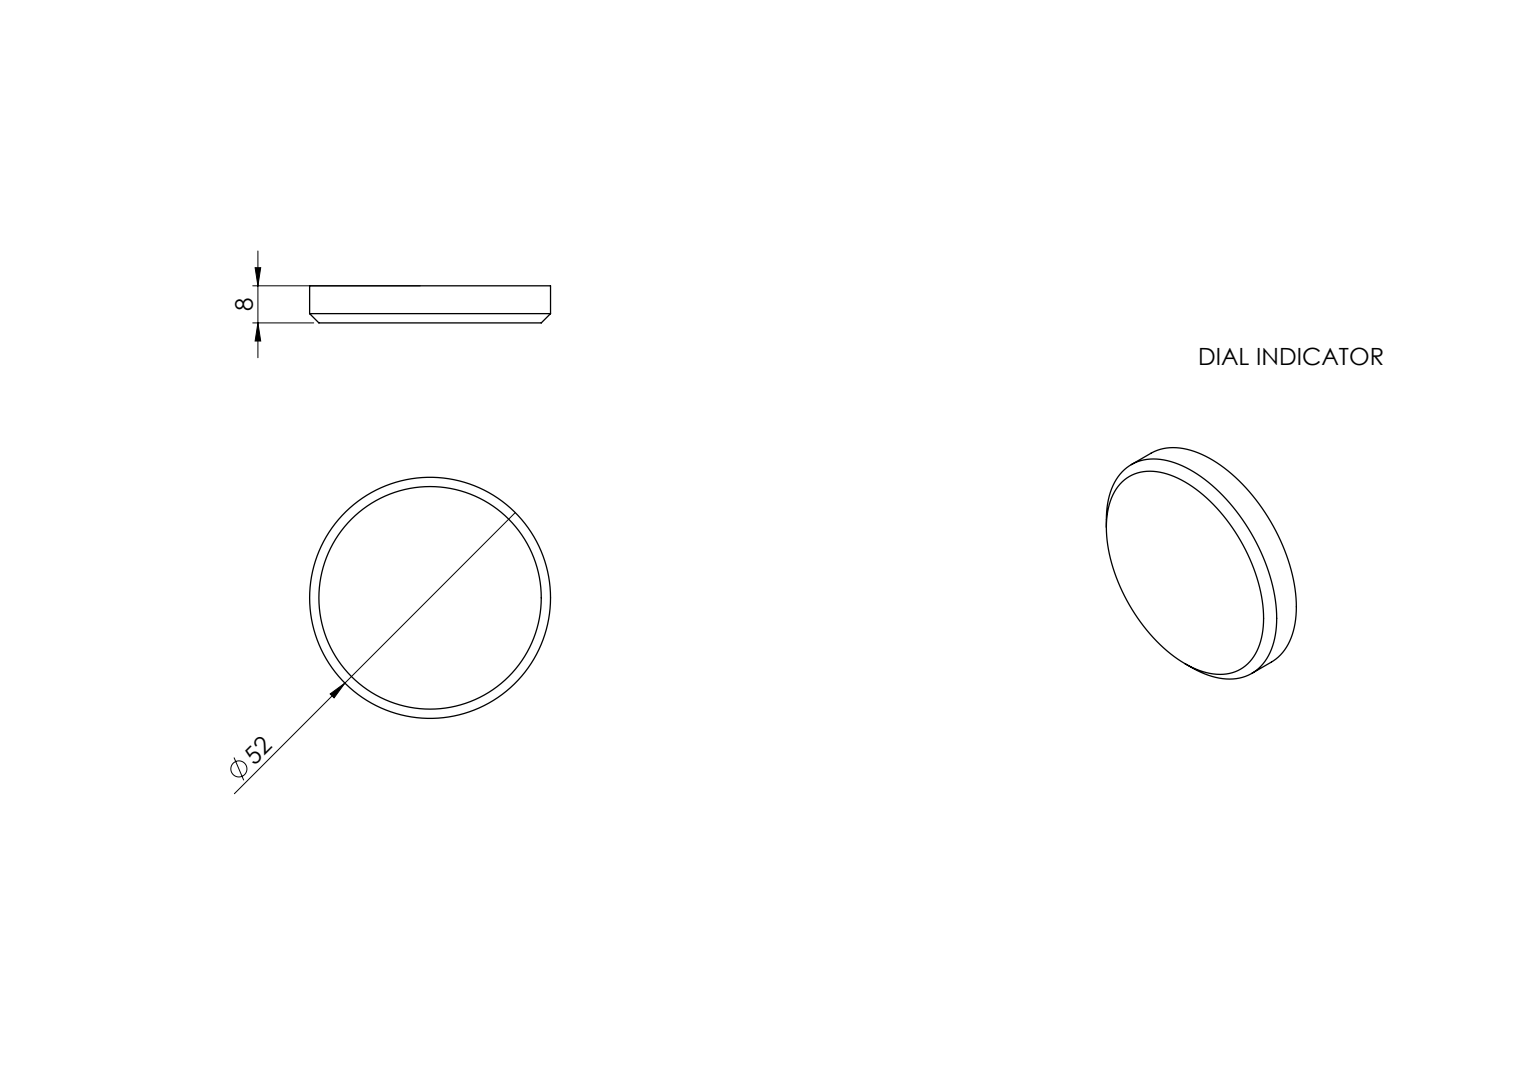
ISO-10303-21;
HEADER;
FILE_DESCRIPTION (('STEP AP214'),
    '1' );
FILE_NAME ('dial indicator.step',
    '2026-10-27T04:40:18',
    ( '' ),
    ( '' ),
    'SwSTEP 2.0',
    'SolidWorks 2026',
    '' );
FILE_SCHEMA (( 'AUTOMOTIVE_DESIGN' ));
ENDSEC;

DATA;
#6=ADVANCED_FACE ( 'NONE', ( #7611 ), #3122, .F. ) ;
#12=DIRECTION ( 'NONE',  ( -1.000000000000000000, 0.000000000000000000, 0.000000000000000000 ) ) ;
#28=DIRECTION ( 'NONE',  ( -1.000000000000000000, 0.000000000000000000, 0.000000000000000000 ) ) ;
#30=LINE ( 'NONE', #3412, #7519 ) ;
#144=CIRCLE ( 'NONE', #2107, 1.000000000000000888 ) ;
#231=DIRECTION ( 'NONE',  ( -1.000000000000000000, 0.000000000000000000, 0.000000000000000000 ) ) ;
#250=DIRECTION ( 'NONE',  ( 1.000000000000000000, 0.000000000000000000, 0.000000000000000000 ) ) ;
#266=DIRECTION ( 'NONE',  ( -0.000000000000000000, -0.000000000000000000, -1.000000000000000000 ) ) ;
#268=DIRECTION ( 'NONE',  ( -1.000000000000000000, 0.000000000000000000, 0.000000000000000000 ) ) ;
#325=EDGE_LOOP ( 'NONE', ( #10518, #10319, #10166, #3050 ) ) ;
#332=LINE ( 'NONE', #9669, #6281 ) ;
#361=ORIENTED_EDGE ( 'NONE', *, *, #10949, .T. ) ;
#401=DIRECTION ( 'NONE',  ( -1.000000000000000000, 0.000000000000000000, 0.000000000000000000 ) ) ;
#435=SURFACE_STYLE_USAGE ( .BOTH. , #2987 ) ;
#461=EDGE_LOOP ( 'NONE', ( #7760, #1425, #10364, #3402 ) ) ;
#484=VERTEX_POINT ( 'NONE', #2961 ) ;
#495=ORIENTED_EDGE ( 'NONE', *, *, #4274, .T. ) ;
#501=CARTESIAN_POINT ( 'NONE',  ( -78.99999999999998579, 11.49999999999999645, 8.000000000000000000 ) ) ;
#506=VERTEX_POINT ( 'NONE', #4670 ) ;
#524=CIRCLE ( 'NONE', #4765, 25.99999999999999645 ) ;
#539=( GEOMETRIC_REPRESENTATION_CONTEXT ( 3 ) GLOBAL_UNCERTAINTY_ASSIGNED_CONTEXT ( ( #6697 ) ) GLOBAL_UNIT_ASSIGNED_CONTEXT ( ( #8208, #6320, #9818 ) ) REPRESENTATION_CONTEXT ( 'NONE', 'WORKASPACE' ) );
#650=( NAMED_UNIT ( * ) PLANE_ANGLE_UNIT ( ) SI_UNIT ( $, .RADIAN. ) );
#658=EDGE_CURVE ( 'NONE', #5256, #1211, #1641, .T. ) ;
#715=ORIENTED_EDGE ( 'NONE', *, *, #4832, .T. ) ;
#780=DIRECTION ( 'NONE',  ( -1.000000000000000000, 0.000000000000000000, 0.000000000000000000 ) ) ;
#782=DIRECTION ( 'NONE',  ( 1.000000000000000000, 0.000000000000000000, 0.000000000000000000 ) ) ;
#839=EDGE_LOOP ( 'NONE', ( #2453, #10131 ) ) ;
#846=DIRECTION ( 'NONE',  ( -0.000000000000000000, -0.000000000000000000, -1.000000000000000000 ) ) ;
#905=AXIS2_PLACEMENT_3D ( 'NONE', #10068, #7575, #3243 ) ;
#911=ADVANCED_FACE ( 'NONE', ( #5426 ), #6787, .F. ) ;
#932=PRODUCT_DEFINITION ( 'UNKNOWN', '', #1061, #2065 ) ;
#973=EDGE_LOOP ( 'NONE', ( #9490, #7582 ) ) ;
#984=LINE ( 'NONE', #3485, #6922 ) ;
#1013=ORIENTED_EDGE ( 'NONE', *, *, #2371, .T. ) ;
#1025=AXIS2_PLACEMENT_3D ( 'NONE', #9855, #4728, #3739 ) ;
#1061=PRODUCT_DEFINITION_FORMATION_WITH_SPECIFIED_SOURCE ( 'ANY', '', #5186, .NOT_KNOWN. ) ;
#1088=CARTESIAN_POINT ( 'NONE',  ( -77.99999999999998579, 0.000000000000000000, 13.00000000000000178 ) ) ;
#1093=CLOSED_SHELL ( 'NONE', ( #1605, #6, #911, #5905, #8098, #4751, #1537, #8268, #4567, #7532, #4371, #5992, #8739, #7906 ) ) ;
#1128=DIRECTION ( 'NONE',  ( 0.8571673013836855759, 1.049727191973305270E-16, -0.5150380737757257466 ) ) ;
#1148=VERTEX_POINT ( 'NONE', #501 ) ;
#1177=EDGE_CURVE ( 'NONE', #4305, #2837, #8754, .T. ) ;
#1195=SHAPE_REPRESENTATION ( 'dial indicator', ( #2307 ), #6386 ) ;
#1205=ORIENTED_EDGE ( 'NONE', *, *, #7217, .F. ) ;
#1211=VERTEX_POINT ( 'NONE', #9579 ) ;
#1218=DIRECTION ( 'NONE',  ( -0.000000000000000000, -0.000000000000000000, -1.000000000000000000 ) ) ;
#1253=VERTEX_POINT ( 'NONE', #10230 ) ;
#1273=EDGE_LOOP ( 'NONE', ( #7281, #1401 ) ) ;
#1306=CARTESIAN_POINT ( 'NONE',  ( -76.99999999999998579, -11.50000000000000711, 8.000000000000000000 ) ) ;
#1309=SHAPE_DEFINITION_REPRESENTATION ( #5090, #1195 ) ;
#1320=FACE_OUTER_BOUND ( 'NONE', #2407, .T. ) ;
#1374=ORIENTED_EDGE ( 'NONE', *, *, #2836, .T. ) ;
#1401=ORIENTED_EDGE ( 'NONE', *, *, #1177, .T. ) ;
#1425=ORIENTED_EDGE ( 'NONE', *, *, #9158, .F. ) ;
#1427=AXIS2_PLACEMENT_3D ( 'NONE', #2719, #9226, #8549 ) ;
#1428=PRESENTATION_STYLE_ASSIGNMENT (( #435 ) ) ;
#1441=DIRECTION ( 'NONE',  ( -0.000000000000000000, -0.000000000000000000, -1.000000000000000000 ) ) ;
#1454=CARTESIAN_POINT ( 'NONE',  ( -77.99999999999998579, -11.50000000000000711, 8.600860617226443239 ) ) ;
#1516=CARTESIAN_POINT ( 'NONE',  ( -78.99999999999998579, 11.49999999999999645, 8.000000000000000000 ) ) ;
#1529=EDGE_LOOP ( 'NONE', ( #4978, #1374, #5395 ) ) ;
#1537=ADVANCED_FACE ( 'NONE', ( #4170 ), #3392, .T. ) ;
#1555=AXIS2_PLACEMENT_3D ( 'NONE', #10106, #4212, #782 ) ;
#1578=VERTEX_POINT ( 'NONE', #3234 ) ;
#1584=COLOUR_RGB ( '',0.8941176470588234615, 0.8941176470588234615, 0.8941176470588234615 ) ;
#1600=DIRECTION ( 'NONE',  ( -0.000000000000000000, -0.000000000000000000, -1.000000000000000000 ) ) ;
#1605=ADVANCED_FACE ( 'NONE', ( #7571 ), #8225, .F. ) ;
#1641=CIRCLE ( 'NONE', #3225, 1.000000000000000888 ) ;
#1646=( NAMED_UNIT ( * ) SI_UNIT ( $, .STERADIAN. ) SOLID_ANGLE_UNIT ( ) );
#1706=DIRECTION ( 'NONE',  ( 1.000000000000000000, 0.000000000000000000, 0.000000000000000000 ) ) ;
#1761=EDGE_LOOP ( 'NONE', ( #3314, #6943, #1013, #10573 ) ) ;
#1777=DIRECTION ( 'NONE',  ( 1.000000000000000000, 0.000000000000000000, 0.000000000000000000 ) ) ;
#1825=VECTOR ( 'NONE', #4554, 1000.000000000000000 ) ;
#1913=ORIENTED_EDGE ( 'NONE', *, *, #7217, .T. ) ;
#1914=DIRECTION ( 'NONE',  ( 0.000000000000000000, 0.000000000000000000, 1.000000000000000000 ) ) ;
#1928=EDGE_CURVE ( 'NONE', #2837, #506, #3848, .T. ) ;
#1938=CARTESIAN_POINT ( 'NONE',  ( -77.99999999999998579, -11.50000000000000711, 8.000000000000000000 ) ) ;
#2015=DIRECTION ( 'NONE',  ( -0.000000000000000000, -0.000000000000000000, -1.000000000000000000 ) ) ;
#2040=( LENGTH_UNIT ( ) NAMED_UNIT ( * ) SI_UNIT ( .MILLI., .METRE. ) );
#2065=PRODUCT_DEFINITION_CONTEXT ( 'detailed design', #3715, 'design' ) ;
#2107=AXIS2_PLACEMENT_3D ( 'NONE', #5307, #266, #3649 ) ;
#2123=DIRECTION ( 'NONE',  ( 1.000000000000000000, 0.000000000000000000, 0.000000000000000000 ) ) ;
#2192=CIRCLE ( 'NONE', #5903, 25.99999999999999645 ) ;
#2257=DIRECTION ( 'NONE',  ( -1.000000000000000000, 0.000000000000000000, 0.000000000000000000 ) ) ;
#2279=DIRECTION ( 'NONE',  ( 0.8571673013836855759, 1.049727191973305270E-16, -0.5150380737757257466 ) ) ;
#2287=DIRECTION ( 'NONE',  ( -1.000000000000000000, 0.000000000000000000, 0.000000000000000000 ) ) ;
#2307=AXIS2_PLACEMENT_3D ( 'NONE', #5193, #3646, #1706 ) ;
#2318=( LENGTH_UNIT ( ) NAMED_UNIT ( * ) SI_UNIT ( .MILLI., .METRE. ) );
#2371=EDGE_CURVE ( 'NONE', #7362, #9156, #6641, .T. ) ;
#2407=EDGE_LOOP ( 'NONE', ( #2965, #10037, #495, #3322 ) ) ;
#2426=CARTESIAN_POINT ( 'NONE',  ( -78.99999999999998579, -11.50000000000000711, 5.000000000000000000 ) ) ;
#2453=ORIENTED_EDGE ( 'NONE', *, *, #10147, .F. ) ;
#2463=FACE_BOUND ( 'NONE', #6963, .T. ) ;
#2473=MECHANICAL_DESIGN_GEOMETRIC_PRESENTATION_REPRESENTATION('',(#7798),#539);
#2508=AXIS2_PLACEMENT_3D ( 'NONE', #10641, #10702, #2257 ) ;
#2561=CARTESIAN_POINT ( 'NONE',  ( -51.99999999999999289, 3.184081677783117796E-15, 5.000000000000000000 ) ) ;
#2613=CONICAL_SURFACE ( 'NONE', #7946, 23.99999999999999289, 0.7853981633974466137 ) ;
#2616=EDGE_LOOP ( 'NONE', ( #5504, #1205, #2931, #6821 ) ) ;
#2661=EDGE_CURVE ( 'NONE', #8992, #506, #3982, .T. ) ;
#2677=DIRECTION ( 'NONE',  ( -0.000000000000000000, -0.000000000000000000, -1.000000000000000000 ) ) ;
#2719=CARTESIAN_POINT ( 'NONE',  ( -77.99999999999998579, 0.000000000000000000, 13.00000000000000178 ) ) ;
#2794=FACE_OUTER_BOUND ( 'NONE', #4485, .T. ) ;
#2827=VECTOR ( 'NONE', #7514, 999.9999999999998863 ) ;
#2836=EDGE_CURVE ( 'NONE', #7251, #5256, #332, .T. ) ;
#2837=VERTEX_POINT ( 'NONE', #3894 ) ;
#2852=CONICAL_SURFACE ( 'NONE', #3364, 1.000000000000000888, 1.029744259999999967 ) ;
#2870=CYLINDRICAL_SURFACE ( 'NONE', #2508, 1.000000000000000888 ) ;
#2915=ORIENTED_EDGE ( 'NONE', *, *, #4504, .T. ) ;
#2931=ORIENTED_EDGE ( 'NONE', *, *, #6699, .T. ) ;
#2939=DIRECTION ( 'NONE',  ( 1.000000000000000000, 0.000000000000000000, -0.000000000000000000 ) ) ;
#2961=CARTESIAN_POINT ( 'NONE',  ( -77.99999999999998579, 11.49999999999999645, 8.600860617226443239 ) ) ;
#2965=ORIENTED_EDGE ( 'NONE', *, *, #7885, .F. ) ;
#2987=SURFACE_SIDE_STYLE ('',( #9874 ) ) ;
#3050=ORIENTED_EDGE ( 'NONE', *, *, #1928, .F. ) ;
#3057=EDGE_CURVE ( 'NONE', #484, #4783, #30, .T. ) ;
#3058=AXIS2_PLACEMENT_3D ( 'NONE', #6518, #9069, #7400 ) ;
#3122=CYLINDRICAL_SURFACE ( 'NONE', #3058, 1.000000000000000888 ) ;
#3136=ORIENTED_EDGE ( 'NONE', *, *, #6578, .F. ) ;
#3180=CIRCLE ( 'NONE', #4398, 25.99999999999999645 ) ;
#3225=AXIS2_PLACEMENT_3D ( 'NONE', #4880, #5720, #10931 ) ;
#3234=CARTESIAN_POINT ( 'NONE',  ( -76.99999999999998579, 11.49999999999999645, 5.000000000000000000 ) ) ;
#3243=DIRECTION ( 'NONE',  ( -1.000000000000000000, 0.000000000000000000, 0.000000000000000000 ) ) ;
#3244=ORIENTED_EDGE ( 'NONE', *, *, #4320, .T. ) ;
#3314=ORIENTED_EDGE ( 'NONE', *, *, #4504, .F. ) ;
#3322=ORIENTED_EDGE ( 'NONE', *, *, #4397, .T. ) ;
#3355=CYLINDRICAL_SURFACE ( 'NONE', #6885, 1.000000000000000888 ) ;
#3364=AXIS2_PLACEMENT_3D ( 'NONE', #9053, #1441, #5707 ) ;
#3392=CYLINDRICAL_SURFACE ( 'NONE', #6453, 25.99999999999999645 ) ;
#3402=ORIENTED_EDGE ( 'NONE', *, *, #2661, .F. ) ;
#3412=CARTESIAN_POINT ( 'NONE',  ( -76.99999999999998579, 11.49999999999999645, 8.000000000000000000 ) ) ;
#3472=EDGE_LOOP ( 'NONE', ( #10356, #8391, #1913 ) ) ;
#3485=CARTESIAN_POINT ( 'NONE',  ( -53.99999999999999289, 2.939152317953647106E-15, 13.00000000000000178 ) ) ;
#3530=CARTESIAN_POINT ( 'NONE',  ( -103.9999999999999858, 0.000000000000000000, 13.00000000000000178 ) ) ;
#3563=ORIENTED_EDGE ( 'NONE', *, *, #8825, .T. ) ;
#3581=CARTESIAN_POINT ( 'NONE',  ( -103.9999999999999858, 0.000000000000000000, 5.000000000000000000 ) ) ;
#3646=DIRECTION ( 'NONE',  ( 0.000000000000000000, 0.000000000000000000, 1.000000000000000000 ) ) ;
#3649=DIRECTION ( 'NONE',  ( -1.000000000000000000, 0.000000000000000000, 0.000000000000000000 ) ) ;
#3695=SHAPE_REPRESENTATION_RELATIONSHIP ( 'NONE' , 'NONE' ,  #1195, #7741 ) ;
#3715=APPLICATION_CONTEXT ( 'automotive_design' ) ;
#3733=CARTESIAN_POINT ( 'NONE',  ( -77.99999999999998579, 11.49999999999999645, 5.000000000000000000 ) ) ;
#3734=CARTESIAN_POINT ( 'NONE',  ( -101.9999999999999858, 0.000000000000000000, 13.00000000000000178 ) ) ;
#3739=DIRECTION ( 'NONE',  ( -1.000000000000000000, 0.000000000000000000, 0.000000000000000000 ) ) ;
#3752=CARTESIAN_POINT ( 'NONE',  ( -77.99999999999998579, -11.50000000000000711, 5.000000000000000000 ) ) ;
#3848=LINE ( 'NONE', #3734, #1825 ) ;
#3877=VECTOR ( 'NONE', #1128, 999.9999999999998863 ) ;
#3894=CARTESIAN_POINT ( 'NONE',  ( -101.9999999999999858, 0.000000000000000000, 13.00000000000000178 ) ) ;
#3982=CIRCLE ( 'NONE', #10167, 25.99999999999999645 ) ;
#4017=CARTESIAN_POINT ( 'NONE',  ( -78.99999999999998579, 11.49999999999999645, 5.000000000000000000 ) ) ;
#4018=DIRECTION ( 'NONE',  ( -0.000000000000000000, -0.000000000000000000, -1.000000000000000000 ) ) ;
#4040=ORIENTED_EDGE ( 'NONE', *, *, #7580, .T. ) ;
#4145=ORIENTED_EDGE ( 'NONE', *, *, #7194, .F. ) ;
#4170=FACE_OUTER_BOUND ( 'NONE', #7161, .T. ) ;
#4212=DIRECTION ( 'NONE',  ( 0.000000000000000000, 0.000000000000000000, 1.000000000000000000 ) ) ;
#4216=CYLINDRICAL_SURFACE ( 'NONE', #6906, 1.000000000000000888 ) ;
#4222=DIRECTION ( 'NONE',  ( -1.000000000000000000, 0.000000000000000000, 0.000000000000000000 ) ) ;
#4237=AXIS2_PLACEMENT_3D ( 'NONE', #3733, #2015, #231 ) ;
#4274=EDGE_CURVE ( 'NONE', #5256, #9156, #10409, .T. ) ;
#4278=CARTESIAN_POINT ( 'NONE',  ( -77.99999999999998579, 0.000000000000000000, 13.00000000000000178 ) ) ;
#4305=VERTEX_POINT ( 'NONE', #7870 ) ;
#4320=EDGE_CURVE ( 'NONE', #5874, #10397, #2192, .T. ) ;
#4371=ADVANCED_FACE ( 'NONE', ( #1320 ), #2870, .F. ) ;
#4397=EDGE_CURVE ( 'NONE', #9156, #7362, #9253, .T. ) ;
#4398=AXIS2_PLACEMENT_3D ( 'NONE', #5923, #5809, #10870 ) ;
#4485=EDGE_LOOP ( 'NONE', ( #9563, #361, #3244, #3136 ) ) ;
#4504=EDGE_CURVE ( 'NONE', #1211, #5256, #7334, .T. ) ;
#4554=DIRECTION ( 'NONE',  ( -0.7071067811865463515, 0.000000000000000000, -0.7071067811865487940 ) ) ;
#4567=ADVANCED_FACE ( 'NONE', ( #2463, #6595, #6648 ), #4961, .F. ) ;
#4581=( NAMED_UNIT ( * ) PLANE_ANGLE_UNIT ( ) SI_UNIT ( $, .RADIAN. ) );
#4622=ORIENTED_EDGE ( 'NONE', *, *, #10648, .F. ) ;
#4670=CARTESIAN_POINT ( 'NONE',  ( -103.9999999999999858, 0.000000000000000000, 10.99999999999999289 ) ) ;
#4721=ORIENTED_EDGE ( 'NONE', *, *, #9877, .T. ) ;
#4728=DIRECTION ( 'NONE',  ( -0.000000000000000000, -0.000000000000000000, -1.000000000000000000 ) ) ;
#4746=ORIENTED_EDGE ( 'NONE', *, *, #2661, .T. ) ;
#4751=ADVANCED_FACE ( 'NONE', ( #2794 ), #6182, .T. ) ;
#4765=AXIS2_PLACEMENT_3D ( 'NONE', #10730, #10774, #2123 ) ;
#4771=DIRECTION ( 'NONE',  ( -0.8571673013836855759, 0.000000000000000000, -0.5150380737757257466 ) ) ;
#4783=VERTEX_POINT ( 'NONE', #6069 ) ;
#4797=LINE ( 'NONE', #4017, #7987 ) ;
#4832=EDGE_CURVE ( 'NONE', #4783, #1148, #6994, .T. ) ;
#4880=CARTESIAN_POINT ( 'NONE',  ( -77.99999999999998579, -11.50000000000000711, 8.000000000000000000 ) ) ;
#4910=STYLED_ITEM('',(#11034),#8606);
#4936=DIRECTION ( 'NONE',  ( -0.000000000000000000, -0.000000000000000000, -1.000000000000000000 ) ) ;
#4941=CONICAL_SURFACE ( 'NONE', #5824, 1.000000000000000888, 1.029744259999999967 ) ;
#4961=PLANE ( 'NONE',  #5872 ) ;
#4975=APPLICATION_CONTEXT ( 'automotive_design' ) ;
#4978=ORIENTED_EDGE ( 'NONE', *, *, #8825, .F. ) ;
#4992=CARTESIAN_POINT ( 'NONE',  ( -77.99999999999998579, -11.50000000000000711, 5.000000000000000000 ) ) ;
#5005=CARTESIAN_POINT ( 'NONE',  ( -77.99999999999998579, 11.49999999999999645, 8.000000000000000000 ) ) ;
#5071=DIRECTION ( 'NONE',  ( -0.000000000000000000, -0.000000000000000000, -1.000000000000000000 ) ) ;
#5089=( GEOMETRIC_REPRESENTATION_CONTEXT ( 3 ) GLOBAL_UNCERTAINTY_ASSIGNED_CONTEXT ( ( #5822 ) ) GLOBAL_UNIT_ASSIGNED_CONTEXT ( ( #2318, #650, #1646 ) ) REPRESENTATION_CONTEXT ( 'NONE', 'WORKASPACE' ) );
#5090=PRODUCT_DEFINITION_SHAPE ( 'NONE', 'NONE',  #932 ) ;
#5147=DIRECTION ( 'NONE',  ( 0.7071067811865463515, 8.659560562354918067E-17, -0.7071067811865487940 ) ) ;
#5186=PRODUCT ( 'dial indicator', 'dial indicator', '', ( #10690 ) ) ;
#5193=CARTESIAN_POINT ( 'NONE',  ( 0.000000000000000000, 0.000000000000000000, 0.000000000000000000 ) ) ;
#5256=VERTEX_POINT ( 'NONE', #9670 ) ;
#5307=CARTESIAN_POINT ( 'NONE',  ( -77.99999999999998579, 11.49999999999999645, 5.000000000000000000 ) ) ;
#5312=LINE ( 'NONE', #8834, #6026 ) ;
#5322=DIRECTION ( 'NONE',  ( -0.000000000000000000, -0.000000000000000000, -1.000000000000000000 ) ) ;
#5335=AXIS2_PLACEMENT_3D ( 'NONE', #3752, #8041, #5638 ) ;
#5359=AXIS2_PLACEMENT_3D ( 'NONE', #8309, #1914, #6022 ) ;
#5395=ORIENTED_EDGE ( 'NONE', *, *, #658, .T. ) ;
#5426=FACE_OUTER_BOUND ( 'NONE', #9487, .T. ) ;
#5485=DIRECTION ( 'NONE',  ( -0.000000000000000000, -0.000000000000000000, -1.000000000000000000 ) ) ;
#5494=CIRCLE ( 'NONE', #7994, 1.000000000000000888 ) ;
#5504=ORIENTED_EDGE ( 'NONE', *, *, #7580, .F. ) ;
#5638=DIRECTION ( 'NONE',  ( -1.000000000000000000, 0.000000000000000000, 0.000000000000000000 ) ) ;
#5670=ORIENTED_EDGE ( 'NONE', *, *, #10147, .T. ) ;
#5681=CARTESIAN_POINT ( 'NONE',  ( -51.99999999999999289, 3.184081677783117796E-15, 10.99999999999999289 ) ) ;
#5690=DIRECTION ( 'NONE',  ( -0.000000000000000000, -0.000000000000000000, -1.000000000000000000 ) ) ;
#5707=DIRECTION ( 'NONE',  ( -1.000000000000000000, 0.000000000000000000, 0.000000000000000000 ) ) ;
#5720=DIRECTION ( 'NONE',  ( -0.000000000000000000, -0.000000000000000000, -1.000000000000000000 ) ) ;
#5809=DIRECTION ( 'NONE',  ( 0.000000000000000000, 0.000000000000000000, 1.000000000000000000 ) ) ;
#5822=UNCERTAINTY_MEASURE_WITH_UNIT (LENGTH_MEASURE( 1.000000000000000082E-05 ), #2318, 'distance_accuracy_value', 'NONE');
#5824=AXIS2_PLACEMENT_3D ( 'NONE', #10387, #5322, #401 ) ;
#5872=AXIS2_PLACEMENT_3D ( 'NONE', #10023, #9976, #8362 ) ;
#5874=VERTEX_POINT ( 'NONE', #2561 ) ;
#5891=AXIS2_PLACEMENT_3D ( 'NONE', #1938, #5485, #268 ) ;
#5897=FACE_OUTER_BOUND ( 'NONE', #1761, .T. ) ;
#5903=AXIS2_PLACEMENT_3D ( 'NONE', #7700, #9584, #250 ) ;
#5905=ADVANCED_FACE ( 'NONE', ( #5897 ), #4216, .F. ) ;
#5923=CARTESIAN_POINT ( 'NONE',  ( -77.99999999999998579, 0.000000000000000000, 5.000000000000000000 ) ) ;
#5992=ADVANCED_FACE ( 'NONE', ( #7788 ), #4941, .F. ) ;
#5996=CARTESIAN_POINT ( 'NONE',  ( -78.99999999999998579, -11.50000000000000711, 5.000000000000000000 ) ) ;
#6022=DIRECTION ( 'NONE',  ( 1.000000000000000000, 0.000000000000000000, 0.000000000000000000 ) ) ;
#6026=VECTOR ( 'NONE', #1218, 1000.000000000000000 ) ;
#6058=DIRECTION ( 'NONE',  ( -1.000000000000000000, 0.000000000000000000, 0.000000000000000000 ) ) ;
#6069=CARTESIAN_POINT ( 'NONE',  ( -76.99999999999998579, 11.49999999999999645, 8.000000000000000000 ) ) ;
#6152=EDGE_CURVE ( 'NONE', #506, #8992, #524, .T. ) ;
#6170=CARTESIAN_POINT ( 'NONE',  ( -51.99999999999999289, 3.184081677783117796E-15, 13.00000000000000178 ) ) ;
#6182=CYLINDRICAL_SURFACE ( 'NONE', #10678, 25.99999999999999645 ) ;
#6227=CARTESIAN_POINT ( 'NONE',  ( -77.99999999999998579, 0.000000000000000000, 10.99999999999999289 ) ) ;
#6281=VECTOR ( 'NONE', #4771, 999.9999999999998863 ) ;
#6320=( NAMED_UNIT ( * ) PLANE_ANGLE_UNIT ( ) SI_UNIT ( $, .RADIAN. ) );
#6356=LINE ( 'NONE', #1306, #3877 ) ;
#6365=CIRCLE ( 'NONE', #1555, 23.99999999999999289 ) ;
#6379=VECTOR ( 'NONE', #7178, 1000.000000000000000 ) ;
#6386=( GEOMETRIC_REPRESENTATION_CONTEXT ( 3 ) GLOBAL_UNCERTAINTY_ASSIGNED_CONTEXT ( ( #8366 ) ) GLOBAL_UNIT_ASSIGNED_CONTEXT ( ( #2040, #4581, #9762 ) ) REPRESENTATION_CONTEXT ( 'NONE', 'WORKASPACE' ) );
#6453=AXIS2_PLACEMENT_3D ( 'NONE', #9187, #4018, #4222 ) ;
#6518=CARTESIAN_POINT ( 'NONE',  ( -77.99999999999998579, 11.49999999999999645, 5.000000000000000000 ) ) ;
#6578=EDGE_CURVE ( 'NONE', #506, #10397, #8711, .T. ) ;
#6595=FACE_BOUND ( 'NONE', #973, .T. ) ;
#6641=CIRCLE ( 'NONE', #7873, 1.000000000000000888 ) ;
#6642=DIRECTION ( 'NONE',  ( -0.000000000000000000, -0.000000000000000000, -1.000000000000000000 ) ) ;
#6648=FACE_OUTER_BOUND ( 'NONE', #839, .T. ) ;
#6673=CARTESIAN_POINT ( 'NONE',  ( -77.99999999999998579, 11.49999999999999645, 8.000000000000000000 ) ) ;
#6697=UNCERTAINTY_MEASURE_WITH_UNIT (LENGTH_MEASURE( 1.000000000000000082E-05 ), #8208, 'distance_accuracy_value', 'NONE');
#6699=EDGE_CURVE ( 'NONE', #1148, #1253, #4797, .T. ) ;
#6752=VECTOR ( 'NONE', #8171, 1000.000000000000000 ) ;
#6758=ORIENTED_EDGE ( 'NONE', *, *, #2836, .F. ) ;
#6784=DIRECTION ( 'NONE',  ( -0.000000000000000000, -0.000000000000000000, -1.000000000000000000 ) ) ;
#6787=CONICAL_SURFACE ( 'NONE', #5891, 1.000000000000000888, 1.029744259999999967 ) ;
#6821=ORIENTED_EDGE ( 'NONE', *, *, #7194, .T. ) ;
#6822=FACE_OUTER_BOUND ( 'NONE', #325, .T. ) ;
#6861=FACE_OUTER_BOUND ( 'NONE', #2616, .T. ) ;
#6885=AXIS2_PLACEMENT_3D ( 'NONE', #10130, #5071, #28 ) ;
#6898=CARTESIAN_POINT ( 'NONE',  ( -77.99999999999998579, -11.50000000000000711, 5.000000000000000000 ) ) ;
#6906=AXIS2_PLACEMENT_3D ( 'NONE', #6898, #2677, #6058 ) ;
#6922=VECTOR ( 'NONE', #5147, 1000.000000000000000 ) ;
#6943=ORIENTED_EDGE ( 'NONE', *, *, #7885, .T. ) ;
#6963=EDGE_LOOP ( 'NONE', ( #4145, #9257 ) ) ;
#6994=CIRCLE ( 'NONE', #1025, 1.000000000000000888 ) ;
#7095=VECTOR ( 'NONE', #7820, 1000.000000000000000 ) ;
#7161=EDGE_LOOP ( 'NONE', ( #8724, #4746, #8965, #5670 ) ) ;
#7178=DIRECTION ( 'NONE',  ( -0.000000000000000000, -0.000000000000000000, -1.000000000000000000 ) ) ;
#7194=EDGE_CURVE ( 'NONE', #1253, #1578, #10275, .T. ) ;
#7215=EDGE_LOOP ( 'NONE', ( #4622, #8272, #715 ) ) ;
#7217=EDGE_CURVE ( 'NONE', #1148, #4783, #5494, .T. ) ;
#7251=VERTEX_POINT ( 'NONE', #1454 ) ;
#7281=ORIENTED_EDGE ( 'NONE', *, *, #9158, .T. ) ;
#7317=FILL_AREA_STYLE ('',( #9037 ) ) ;
#7332=CARTESIAN_POINT ( 'NONE',  ( -76.99999999999998579, -11.50000000000000711, 5.000000000000000000 ) ) ;
#7334=CIRCLE ( 'NONE', #905, 1.000000000000000888 ) ;
#7362=VERTEX_POINT ( 'NONE', #8129 ) ;
#7387=EDGE_CURVE ( 'NONE', #4305, #8992, #984, .T. ) ;
#7400=DIRECTION ( 'NONE',  ( -1.000000000000000000, 0.000000000000000000, 0.000000000000000000 ) ) ;
#7413=ORIENTED_EDGE ( 'NONE', *, *, #6699, .F. ) ;
#7440=LINE ( 'NONE', #7332, #6752 ) ;
#7514=DIRECTION ( 'NONE',  ( -0.8571673013836855759, 0.000000000000000000, -0.5150380737757257466 ) ) ;
#7519=VECTOR ( 'NONE', #2279, 999.9999999999998863 ) ;
#7532=ADVANCED_FACE ( 'NONE', ( #7555 ), #10819, .T. ) ;
#7555=FACE_OUTER_BOUND ( 'NONE', #461, .T. ) ;
#7571=FACE_OUTER_BOUND ( 'NONE', #7215, .T. ) ;
#7575=DIRECTION ( 'NONE',  ( -0.000000000000000000, -0.000000000000000000, -1.000000000000000000 ) ) ;
#7580=EDGE_CURVE ( 'NONE', #4783, #1578, #5312, .T. ) ;
#7582=ORIENTED_EDGE ( 'NONE', *, *, #2371, .F. ) ;
#7611=FACE_OUTER_BOUND ( 'NONE', #9630, .T. ) ;
#7700=CARTESIAN_POINT ( 'NONE',  ( -77.99999999999998579, 0.000000000000000000, 5.000000000000000000 ) ) ;
#7741=ADVANCED_BREP_SHAPE_REPRESENTATION ( '', ( #8606, #2307 ), #6386 ) ;
#7760=ORIENTED_EDGE ( 'NONE', *, *, #7387, .F. ) ;
#7788=FACE_OUTER_BOUND ( 'NONE', #1529, .T. ) ;
#7798=STYLED_ITEM ( 'NONE', ( #1428 ), #7741 ) ;
#7820=DIRECTION ( 'NONE',  ( -0.000000000000000000, -0.000000000000000000, -1.000000000000000000 ) ) ;
#7854=DIRECTION ( 'NONE',  ( -1.000000000000000000, 0.000000000000000000, 0.000000000000000000 ) ) ;
#7870=CARTESIAN_POINT ( 'NONE',  ( -53.99999999999999289, 3.061616997868382254E-15, 13.00000000000000178 ) ) ;
#7873=AXIS2_PLACEMENT_3D ( 'NONE', #4992, #6784, #780 ) ;
#7885=EDGE_CURVE ( 'NONE', #1211, #7362, #7440, .T. ) ;
#7906=ADVANCED_FACE ( 'NONE', ( #8273 ), #2852, .F. ) ;
#7946=AXIS2_PLACEMENT_3D ( 'NONE', #10924, #8430, #8378 ) ;
#7987=VECTOR ( 'NONE', #6642, 1000.000000000000000 ) ;
#7994=AXIS2_PLACEMENT_3D ( 'NONE', #6673, #4936, #2287 ) ;
#8041=DIRECTION ( 'NONE',  ( -0.000000000000000000, -0.000000000000000000, -1.000000000000000000 ) ) ;
#8048=AXIS2_PLACEMENT_3D ( 'NONE', #5005, #5690, #12 ) ;
#8098=ADVANCED_FACE ( 'NONE', ( #6822 ), #2613, .T. ) ;
#8129=CARTESIAN_POINT ( 'NONE',  ( -76.99999999999998579, -11.50000000000000711, 5.000000000000000000 ) ) ;
#8171=DIRECTION ( 'NONE',  ( -0.000000000000000000, -0.000000000000000000, -1.000000000000000000 ) ) ;
#8208=( LENGTH_UNIT ( ) NAMED_UNIT ( * ) SI_UNIT ( .MILLI., .METRE. ) );
#8225=CONICAL_SURFACE ( 'NONE', #8048, 1.000000000000000888, 1.029744259999999967 ) ;
#8268=ADVANCED_FACE ( 'NONE', ( #8882 ), #9534, .T. ) ;
#8272=ORIENTED_EDGE ( 'NONE', *, *, #3057, .T. ) ;
#8273=FACE_OUTER_BOUND ( 'NONE', #3472, .T. ) ;
#8309=CARTESIAN_POINT ( 'NONE',  ( -77.99999999999998579, 0.000000000000000000, 13.00000000000000178 ) ) ;
#8362=DIRECTION ( 'NONE',  ( 1.000000000000000000, 0.000000000000000000, -0.000000000000000000 ) ) ;
#8366=UNCERTAINTY_MEASURE_WITH_UNIT (LENGTH_MEASURE( 1.000000000000000082E-05 ), #2040, 'distance_accuracy_value', 'NONE');
#8378=DIRECTION ( 'NONE',  ( -1.000000000000000000, 0.000000000000000000, 0.000000000000000000 ) ) ;
#8391=ORIENTED_EDGE ( 'NONE', *, *, #10648, .T. ) ;
#8430=DIRECTION ( 'NONE',  ( 0.000000000000000000, 0.000000000000000000, -1.000000000000000000 ) ) ;
#8499=DIRECTION ( 'NONE',  ( 0.000000000000000000, 0.000000000000000000, -1.000000000000000000 ) ) ;
#8549=DIRECTION ( 'NONE',  ( -1.000000000000000000, 0.000000000000000000, 0.000000000000000000 ) ) ;
#8606=MANIFOLD_SOLID_BREP ( 'AdvancedHole1', #1093 ) ;
#8711=LINE ( 'NONE', #3530, #7095 ) ;
#8724=ORIENTED_EDGE ( 'NONE', *, *, #10949, .F. ) ;
#8739=ADVANCED_FACE ( 'NONE', ( #6861 ), #3355, .F. ) ;
#8754=CIRCLE ( 'NONE', #5359, 23.99999999999999289 ) ;
#8825=EDGE_CURVE ( 'NONE', #7251, #1211, #6356, .T. ) ;
#8834=CARTESIAN_POINT ( 'NONE',  ( -76.99999999999998579, 11.49999999999999645, 5.000000000000000000 ) ) ;
#8882=FACE_OUTER_BOUND ( 'NONE', #1273, .T. ) ;
#8965=ORIENTED_EDGE ( 'NONE', *, *, #6578, .T. ) ;
#8992=VERTEX_POINT ( 'NONE', #5681 ) ;
#9037=FILL_AREA_STYLE_COLOUR ( '', #1584 ) ;
#9053=CARTESIAN_POINT ( 'NONE',  ( -77.99999999999998579, 11.49999999999999645, 8.000000000000000000 ) ) ;
#9069=DIRECTION ( 'NONE',  ( -0.000000000000000000, -0.000000000000000000, -1.000000000000000000 ) ) ;
#9129=LINE ( 'NONE', #1516, #2827 ) ;
#9156=VERTEX_POINT ( 'NONE', #5996 ) ;
#9158=EDGE_CURVE ( 'NONE', #2837, #4305, #6365, .T. ) ;
#9182=MECHANICAL_DESIGN_GEOMETRIC_PRESENTATION_REPRESENTATION('',(#4910),#5089);
#9187=CARTESIAN_POINT ( 'NONE',  ( -77.99999999999998579, 0.000000000000000000, 13.00000000000000178 ) ) ;
#9226=DIRECTION ( 'NONE',  ( 0.000000000000000000, 0.000000000000000000, -1.000000000000000000 ) ) ;
#9253=CIRCLE ( 'NONE', #5335, 1.000000000000000888 ) ;
#9257=ORIENTED_EDGE ( 'NONE', *, *, #9877, .F. ) ;
#9272=VECTOR ( 'NONE', #1600, 1000.000000000000000 ) ;
#9487=EDGE_LOOP ( 'NONE', ( #6758, #3563, #2915 ) ) ;
#9490=ORIENTED_EDGE ( 'NONE', *, *, #4397, .F. ) ;
#9534=PLANE ( 'NONE',  #10598 ) ;
#9563=ORIENTED_EDGE ( 'NONE', *, *, #6152, .T. ) ;
#9579=CARTESIAN_POINT ( 'NONE',  ( -76.99999999999998579, -11.50000000000000711, 8.000000000000000000 ) ) ;
#9584=DIRECTION ( 'NONE',  ( 0.000000000000000000, 0.000000000000000000, 1.000000000000000000 ) ) ;
#9616=LINE ( 'NONE', #6170, #6379 ) ;
#9630=EDGE_LOOP ( 'NONE', ( #9865, #4040, #4721, #7413 ) ) ;
#9669=CARTESIAN_POINT ( 'NONE',  ( -78.99999999999998579, -11.50000000000000711, 8.000000000000000000 ) ) ;
#9670=CARTESIAN_POINT ( 'NONE',  ( -78.99999999999998579, -11.50000000000000711, 8.000000000000000000 ) ) ;
#9762=( NAMED_UNIT ( * ) SI_UNIT ( $, .STERADIAN. ) SOLID_ANGLE_UNIT ( ) );
#9818=( NAMED_UNIT ( * ) SI_UNIT ( $, .STERADIAN. ) SOLID_ANGLE_UNIT ( ) );
#9855=CARTESIAN_POINT ( 'NONE',  ( -77.99999999999998579, 11.49999999999999645, 8.000000000000000000 ) ) ;
#9865=ORIENTED_EDGE ( 'NONE', *, *, #4832, .F. ) ;
#9874=SURFACE_STYLE_FILL_AREA ( #7317 ) ;
#9877=EDGE_CURVE ( 'NONE', #1578, #1253, #144, .T. ) ;
#9976=DIRECTION ( 'NONE',  ( 0.000000000000000000, 0.000000000000000000, 1.000000000000000000 ) ) ;
#10023=CARTESIAN_POINT ( 'NONE',  ( -77.99999999999998579, 0.000000000000000000, 5.000000000000000000 ) ) ;
#10037=ORIENTED_EDGE ( 'NONE', *, *, #658, .F. ) ;
#10068=CARTESIAN_POINT ( 'NONE',  ( -77.99999999999998579, -11.50000000000000711, 8.000000000000000000 ) ) ;
#10106=CARTESIAN_POINT ( 'NONE',  ( -77.99999999999998579, 0.000000000000000000, 13.00000000000000178 ) ) ;
#10130=CARTESIAN_POINT ( 'NONE',  ( -77.99999999999998579, 11.49999999999999645, 5.000000000000000000 ) ) ;
#10131=ORIENTED_EDGE ( 'NONE', *, *, #4320, .F. ) ;
#10147=EDGE_CURVE ( 'NONE', #10397, #5874, #3180, .T. ) ;
#10166=ORIENTED_EDGE ( 'NONE', *, *, #6152, .F. ) ;
#10167=AXIS2_PLACEMENT_3D ( 'NONE', #6227, #8499, #1777 ) ;
#10230=CARTESIAN_POINT ( 'NONE',  ( -78.99999999999998579, 11.49999999999999645, 5.000000000000000000 ) ) ;
#10275=CIRCLE ( 'NONE', #4237, 1.000000000000000888 ) ;
#10319=ORIENTED_EDGE ( 'NONE', *, *, #7387, .T. ) ;
#10356=ORIENTED_EDGE ( 'NONE', *, *, #3057, .F. ) ;
#10364=ORIENTED_EDGE ( 'NONE', *, *, #1928, .T. ) ;
#10387=CARTESIAN_POINT ( 'NONE',  ( -77.99999999999998579, -11.50000000000000711, 8.000000000000000000 ) ) ;
#10397=VERTEX_POINT ( 'NONE', #3581 ) ;
#10409=LINE ( 'NONE', #2426, #9272 ) ;
#10518=ORIENTED_EDGE ( 'NONE', *, *, #1177, .F. ) ;
#10540=DIRECTION ( 'NONE',  ( 0.000000000000000000, 0.000000000000000000, 1.000000000000000000 ) ) ;
#10573=ORIENTED_EDGE ( 'NONE', *, *, #4274, .F. ) ;
#10598=AXIS2_PLACEMENT_3D ( 'NONE', #1088, #10540, #2939 ) ;
#10641=CARTESIAN_POINT ( 'NONE',  ( -77.99999999999998579, -11.50000000000000711, 5.000000000000000000 ) ) ;
#10648=EDGE_CURVE ( 'NONE', #484, #1148, #9129, .T. ) ;
#10678=AXIS2_PLACEMENT_3D ( 'NONE', #4278, #846, #7854 ) ;
#10690=PRODUCT_CONTEXT ( 'NONE', #4975, 'mechanical' ) ;
#10702=DIRECTION ( 'NONE',  ( -0.000000000000000000, -0.000000000000000000, -1.000000000000000000 ) ) ;
#10730=CARTESIAN_POINT ( 'NONE',  ( -77.99999999999998579, 0.000000000000000000, 10.99999999999999289 ) ) ;
#10774=DIRECTION ( 'NONE',  ( 0.000000000000000000, 0.000000000000000000, -1.000000000000000000 ) ) ;
#10819=CONICAL_SURFACE ( 'NONE', #1427, 23.99999999999999289, 0.7853981633974466137 ) ;
#10870=DIRECTION ( 'NONE',  ( 1.000000000000000000, 0.000000000000000000, 0.000000000000000000 ) ) ;
#10924=CARTESIAN_POINT ( 'NONE',  ( -77.99999999999998579, 0.000000000000000000, 13.00000000000000178 ) ) ;
#10931=DIRECTION ( 'NONE',  ( -1.000000000000000000, 0.000000000000000000, 0.000000000000000000 ) ) ;
#10949=EDGE_CURVE ( 'NONE', #8992, #5874, #9616, .T. ) ;
#11028=COLOUR_RGB('Off White',0.89,0.88,0.83);
#11029=FILL_AREA_STYLE_COLOUR('',#11028);
#11030=FILL_AREA_STYLE('',(#11029));
#11031=SURFACE_STYLE_FILL_AREA(#11030);
#11032=SURFACE_SIDE_STYLE('',(#11031));
#11033=SURFACE_STYLE_USAGE(.BOTH.,#11032);
#11034=PRESENTATION_STYLE_ASSIGNMENT((#11033));
ENDSEC;
END-ISO-10303-21;
